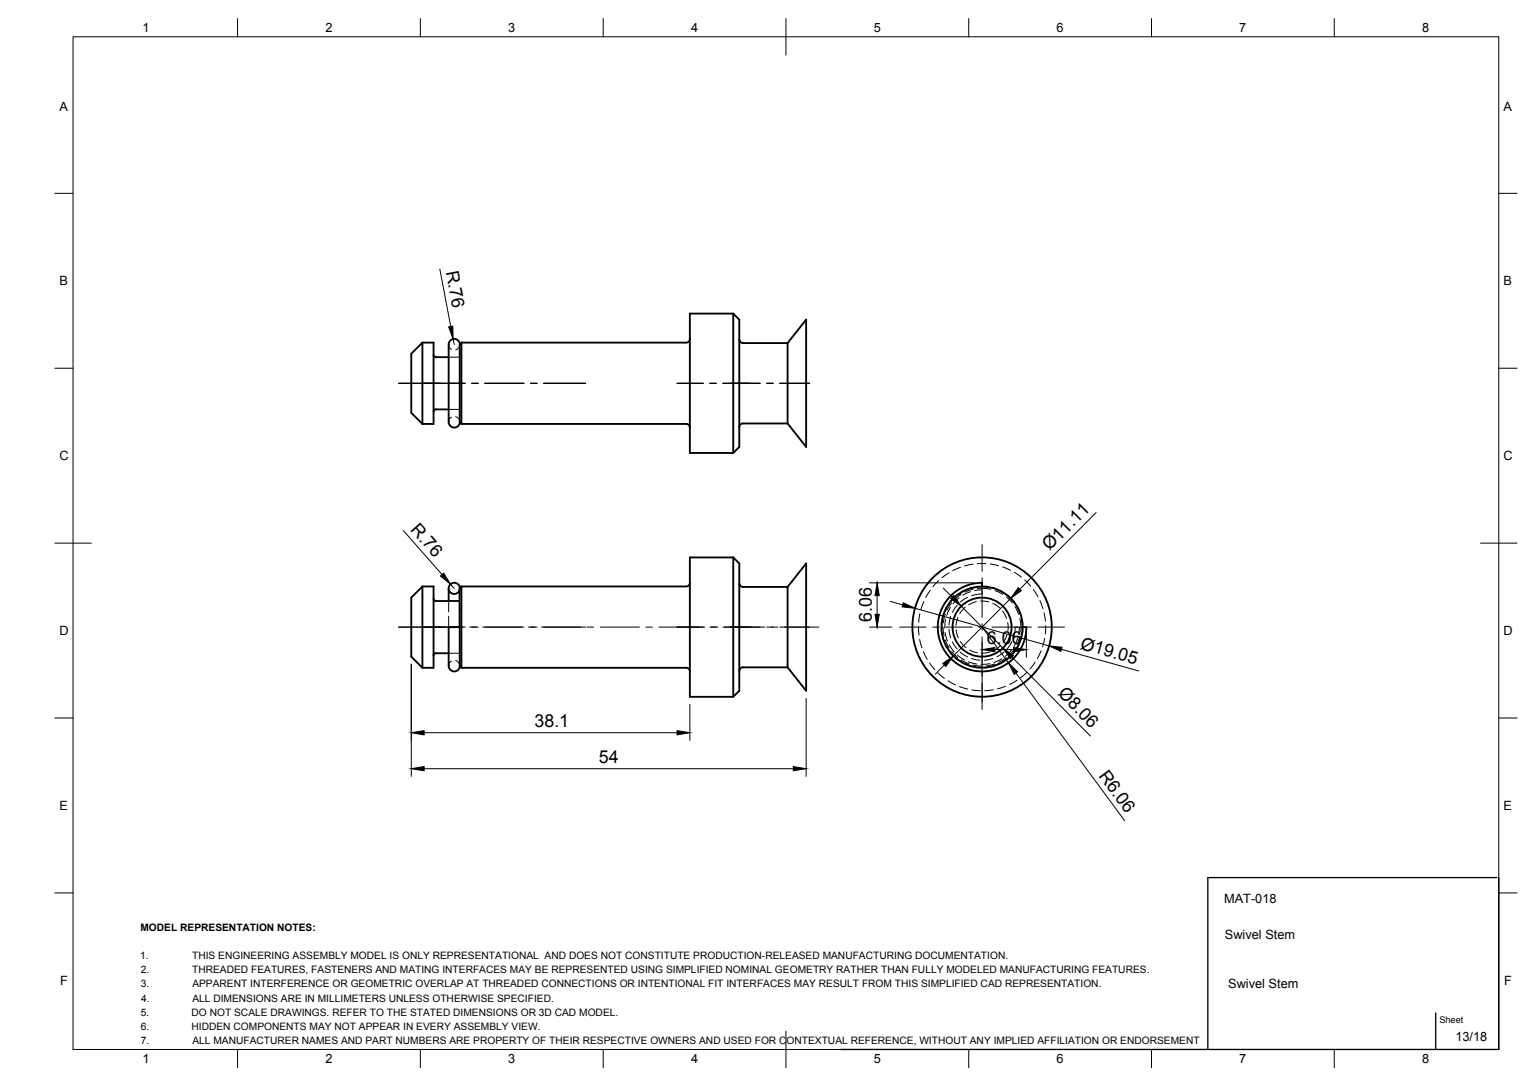
ISO-10303-21;
HEADER;
/* Generated by software containing ST-Developer
 * from STEP Tools, Inc. (www.steptools.com) 
 */

FILE_DESCRIPTION(
/* description */ ('STEP AP214'),
/* implementation_level */ '2;1');

FILE_NAME(
/* name */ 'Swivel Stem.step',
/* time_stamp */ '2026-11-14T06:16:09-08:00',
/* author */ (''),
/* organization */ (''),
/* preprocessor_version */ 'ST-DEVELOPER v20.2',
/* originating_system */ 'Autodesk Translation Framework v15.17.0.0',
/* authorisation */ '');

FILE_SCHEMA (('AUTOMOTIVE_DESIGN { 1 0 10303 214 3 1 1 }'));
ENDSEC;

DATA;
#10=MECHANICAL_DESIGN_GEOMETRIC_PRESENTATION_REPRESENTATION('',(#357),#18006);
#137=CONICAL_SURFACE('',#10642,5.30225,0.78539816339744);
#138=CONICAL_SURFACE('',#10645,4.03225,0.785398163397449);
#139=CONICAL_SURFACE('',#10665,9.525,0.785398163397447);
#140=CONICAL_SURFACE('',#10673,5.4991,0.899938860194128);
#248=TOROIDAL_SURFACE('',#10636,5.2959,0.762);
#249=TOROIDAL_SURFACE('',#10650,3.8862,0.3175);
#250=TOROIDAL_SURFACE('',#10658,6.06425,0.508);
#251=TOROIDAL_SURFACE('',#10667,6.0071,0.508);
#325=SHAPE_REPRESENTATION_RELATIONSHIP('SRR','None',#18083,#341);
#341=ADVANCED_BREP_SHAPE_REPRESENTATION('',(#373),#18000);
#357=STYLED_ITEM('',(#18170),#373);
#373=MANIFOLD_SOLID_BREP('Body1',#9566);
#478=FACE_BOUND('',#2020,.T.);
#479=FACE_BOUND('',#2022,.T.);
#480=FACE_BOUND('',#2024,.T.);
#481=FACE_BOUND('',#2027,.T.);
#805=PLANE('',#10675);
#806=PLANE('',#10676);
#807=PLANE('',#10677);
#808=PLANE('',#10678);
#809=PLANE('',#10679);
#810=PLANE('',#10680);
#811=PLANE('',#10681);
#812=PLANE('',#10682);
#1328=FACE_OUTER_BOUND('',#2003,.T.);
#1329=FACE_OUTER_BOUND('',#2004,.T.);
#1330=FACE_OUTER_BOUND('',#2005,.T.);
#1331=FACE_OUTER_BOUND('',#2006,.T.);
#1332=FACE_OUTER_BOUND('',#2007,.T.);
#1333=FACE_OUTER_BOUND('',#2008,.T.);
#1334=FACE_OUTER_BOUND('',#2009,.T.);
#1335=FACE_OUTER_BOUND('',#2010,.T.);
#1336=FACE_OUTER_BOUND('',#2011,.T.);
#1337=FACE_OUTER_BOUND('',#2012,.T.);
#1338=FACE_OUTER_BOUND('',#2013,.T.);
#1339=FACE_OUTER_BOUND('',#2014,.T.);
#1340=FACE_OUTER_BOUND('',#2015,.T.);
#1341=FACE_OUTER_BOUND('',#2016,.T.);
#1342=FACE_OUTER_BOUND('',#2017,.T.);
#1343=FACE_OUTER_BOUND('',#2018,.T.);
#1344=FACE_OUTER_BOUND('',#2019,.T.);
#1345=FACE_OUTER_BOUND('',#2021,.T.);
#1346=FACE_OUTER_BOUND('',#2023,.T.);
#1347=FACE_OUTER_BOUND('',#2025,.T.);
#1348=FACE_OUTER_BOUND('',#2026,.T.);
#2003=EDGE_LOOP('',(#8466,#8467,#8468,#8469,#8470));
#2004=EDGE_LOOP('',(#8471,#8472,#8473,#8474,#8475,#8476,#8477,#8478));
#2005=EDGE_LOOP('',(#8479,#8480,#8481,#8482));
#2006=EDGE_LOOP('',(#8483,#8484,#8485,#8486));
#2007=EDGE_LOOP('',(#8487,#8488,#8489,#8490));
#2008=EDGE_LOOP('',(#8491,#8492,#8493,#8494));
#2009=EDGE_LOOP('',(#8495,#8496,#8497,#8498));
#2010=EDGE_LOOP('',(#8499,#8500,#8501,#8502));
#2011=EDGE_LOOP('',(#8503,#8504,#8505,#8506,#8507));
#2012=EDGE_LOOP('',(#8508,#8509,#8510,#8511,#8512));
#2013=EDGE_LOOP('',(#8513,#8514,#8515,#8516));
#2014=EDGE_LOOP('',(#8517,#8518,#8519,#8520));
#2015=EDGE_LOOP('',(#8521,#8522,#8523,#8524));
#2016=EDGE_LOOP('',(#8525,#8526,#8527));
#2017=EDGE_LOOP('',(#8528,#8529,#8530));
#2018=EDGE_LOOP('',(#8531));
#2019=EDGE_LOOP('',(#8532));
#2020=EDGE_LOOP('',(#8533));
#2021=EDGE_LOOP('',(#8534));
#2022=EDGE_LOOP('',(#8535));
#2023=EDGE_LOOP('',(#8536));
#2024=EDGE_LOOP('',(#8537));
#2025=EDGE_LOOP('',(#8538));
#2026=EDGE_LOOP('',(#8539,#8540,#8541,#8542));
#2027=EDGE_LOOP('',(#8543));
#2779=LINE('',#17587,#3503);
#2780=LINE('',#17589,#3504);
#2781=LINE('',#17592,#3505);
#2782=LINE('',#17597,#3506);
#2783=LINE('',#17602,#3507);
#2784=LINE('',#17612,#3508);
#2785=LINE('',#17616,#3509);
#2786=LINE('',#17627,#3510);
#2787=LINE('',#17631,#3511);
#2788=LINE('',#17642,#3512);
#2789=LINE('',#17646,#3513);
#2790=LINE('',#17648,#3514);
#2791=LINE('',#17650,#3515);
#3503=VECTOR('',#13314,5.30225);
#3504=VECTOR('',#13315,1000.);
#3505=VECTOR('',#13318,1000.);
#3506=VECTOR('',#13323,4.03225);
#3507=VECTOR('',#13330,5.55625);
#3508=VECTOR('',#13343,3.5687);
#3509=VECTOR('',#13348,5.55625);
#3510=VECTOR('',#13361,9.525);
#3511=VECTOR('',#13366,9.525);
#3512=VECTOR('',#13381,5.4991);
#3513=VECTOR('',#13386,5.4991);
#3514=VECTOR('',#13389,1000.);
#3515=VECTOR('',#13392,1000.);
#3903=CIRCLE('',#10637,0.762);
#3904=CIRCLE('',#10638,5.32701449118557);
#3905=CIRCLE('',#10639,5.32701449118557);
#3906=CIRCLE('',#10640,0.762);
#3907=CIRCLE('',#10641,5.10079889800413);
#3908=CIRCLE('',#10643,5.55625);
#3909=CIRCLE('',#10644,5.30225);
#3910=CIRCLE('',#10646,5.55625);
#3911=CIRCLE('',#10647,4.03225);
#3912=CIRCLE('',#10649,5.55625);
#3913=CIRCLE('',#10651,3.5687);
#3914=CIRCLE('',#10652,0.3175);
#3915=CIRCLE('',#10653,3.8862);
#3916=CIRCLE('',#10655,3.5687);
#3917=CIRCLE('',#10657,5.55625);
#3918=CIRCLE('',#10659,6.06425);
#3919=CIRCLE('',#10660,0.508);
#3920=CIRCLE('',#10662,9.525);
#3921=CIRCLE('',#10663,9.525);
#3922=CIRCLE('',#10664,9.525);
#3923=CIRCLE('',#10666,8.6995);
#3924=CIRCLE('',#10668,5.4991);
#3925=CIRCLE('',#10669,0.508);
#3926=CIRCLE('',#10670,6.0071);
#3927=CIRCLE('',#10672,5.4991);
#3928=CIRCLE('',#10674,8.6995);
#4716=VERTEX_POINT('',#17574);
#4717=VERTEX_POINT('',#17575);
#4718=VERTEX_POINT('',#17577);
#4719=VERTEX_POINT('',#17579);
#4720=VERTEX_POINT('',#17581);
#4721=VERTEX_POINT('',#17585);
#4722=VERTEX_POINT('',#17588);
#4723=VERTEX_POINT('',#17590);
#4724=VERTEX_POINT('',#17594);
#4725=VERTEX_POINT('',#17596);
#4726=VERTEX_POINT('',#17600);
#4727=VERTEX_POINT('',#17604);
#4728=VERTEX_POINT('',#17606);
#4729=VERTEX_POINT('',#17610);
#4730=VERTEX_POINT('',#17614);
#4731=VERTEX_POINT('',#17618);
#4732=VERTEX_POINT('',#17622);
#4733=VERTEX_POINT('',#17623);
#4734=VERTEX_POINT('',#17626);
#4735=VERTEX_POINT('',#17630);
#4736=VERTEX_POINT('',#17634);
#4737=VERTEX_POINT('',#17636);
#4738=VERTEX_POINT('',#17640);
#4739=VERTEX_POINT('',#17644);
#5981=EDGE_CURVE('',#4716,#4717,#3903,.T.);
#5982=EDGE_CURVE('',#4718,#4716,#3904,.T.);
#5983=EDGE_CURVE('',#4719,#4718,#3905,.T.);
#5984=EDGE_CURVE('',#4719,#4720,#3906,.T.);
#5985=EDGE_CURVE('',#4717,#4720,#3907,.T.);
#5986=EDGE_CURVE('',#4721,#4721,#3908,.T.);
#5987=EDGE_CURVE('',#4721,#4718,#2779,.T.);
#5988=EDGE_CURVE('',#4716,#4722,#2780,.T.);
#5989=EDGE_CURVE('',#4722,#4723,#3909,.T.);
#5990=EDGE_CURVE('',#4719,#4723,#2781,.T.);
#5991=EDGE_CURVE('',#4724,#4724,#3910,.T.);
#5992=EDGE_CURVE('',#4724,#4725,#2782,.T.);
#5993=EDGE_CURVE('',#4725,#4725,#3911,.T.);
#5994=EDGE_CURVE('',#4726,#4726,#3912,.T.);
#5995=EDGE_CURVE('',#4726,#4724,#2783,.T.);
#5996=EDGE_CURVE('',#4727,#4727,#3913,.T.);
#5997=EDGE_CURVE('',#4727,#4728,#3914,.T.);
#5998=EDGE_CURVE('',#4728,#4728,#3915,.T.);
#5999=EDGE_CURVE('',#4729,#4729,#3916,.T.);
#6000=EDGE_CURVE('',#4729,#4727,#2784,.T.);
#6001=EDGE_CURVE('',#4730,#4730,#3917,.T.);
#6002=EDGE_CURVE('',#4730,#4721,#2785,.T.);
#6003=EDGE_CURVE('',#4731,#4731,#3918,.T.);
#6004=EDGE_CURVE('',#4731,#4730,#3919,.T.);
#6005=EDGE_CURVE('',#4732,#4733,#3920,.T.);
#6006=EDGE_CURVE('',#4733,#4732,#3921,.T.);
#6007=EDGE_CURVE('',#4733,#4734,#2786,.T.);
#6008=EDGE_CURVE('',#4734,#4734,#3922,.T.);
#6009=EDGE_CURVE('',#4732,#4735,#2787,.T.);
#6010=EDGE_CURVE('',#4735,#4735,#3923,.T.);
#6011=EDGE_CURVE('',#4736,#4736,#3924,.T.);
#6012=EDGE_CURVE('',#4736,#4737,#3925,.T.);
#6013=EDGE_CURVE('',#4737,#4737,#3926,.T.);
#6014=EDGE_CURVE('',#4738,#4738,#3927,.T.);
#6015=EDGE_CURVE('',#4738,#4736,#2788,.T.);
#6016=EDGE_CURVE('',#4739,#4739,#3928,.T.);
#6017=EDGE_CURVE('',#4739,#4738,#2789,.T.);
#6018=EDGE_CURVE('',#4722,#4717,#2790,.T.);
#6019=EDGE_CURVE('',#4723,#4720,#2791,.T.);
#8466=ORIENTED_EDGE('',*,*,#5981,.F.);
#8467=ORIENTED_EDGE('',*,*,#5982,.F.);
#8468=ORIENTED_EDGE('',*,*,#5983,.F.);
#8469=ORIENTED_EDGE('',*,*,#5984,.T.);
#8470=ORIENTED_EDGE('',*,*,#5985,.F.);
#8471=ORIENTED_EDGE('',*,*,#5986,.F.);
#8472=ORIENTED_EDGE('',*,*,#5987,.T.);
#8473=ORIENTED_EDGE('',*,*,#5982,.T.);
#8474=ORIENTED_EDGE('',*,*,#5988,.T.);
#8475=ORIENTED_EDGE('',*,*,#5989,.T.);
#8476=ORIENTED_EDGE('',*,*,#5990,.F.);
#8477=ORIENTED_EDGE('',*,*,#5983,.T.);
#8478=ORIENTED_EDGE('',*,*,#5987,.F.);
#8479=ORIENTED_EDGE('',*,*,#5991,.F.);
#8480=ORIENTED_EDGE('',*,*,#5992,.T.);
#8481=ORIENTED_EDGE('',*,*,#5993,.T.);
#8482=ORIENTED_EDGE('',*,*,#5992,.F.);
#8483=ORIENTED_EDGE('',*,*,#5994,.F.);
#8484=ORIENTED_EDGE('',*,*,#5995,.T.);
#8485=ORIENTED_EDGE('',*,*,#5991,.T.);
#8486=ORIENTED_EDGE('',*,*,#5995,.F.);
#8487=ORIENTED_EDGE('',*,*,#5996,.F.);
#8488=ORIENTED_EDGE('',*,*,#5997,.T.);
#8489=ORIENTED_EDGE('',*,*,#5998,.T.);
#8490=ORIENTED_EDGE('',*,*,#5997,.F.);
#8491=ORIENTED_EDGE('',*,*,#5999,.F.);
#8492=ORIENTED_EDGE('',*,*,#6000,.T.);
#8493=ORIENTED_EDGE('',*,*,#5996,.T.);
#8494=ORIENTED_EDGE('',*,*,#6000,.F.);
#8495=ORIENTED_EDGE('',*,*,#6001,.F.);
#8496=ORIENTED_EDGE('',*,*,#6002,.T.);
#8497=ORIENTED_EDGE('',*,*,#5986,.T.);
#8498=ORIENTED_EDGE('',*,*,#6002,.F.);
#8499=ORIENTED_EDGE('',*,*,#6003,.F.);
#8500=ORIENTED_EDGE('',*,*,#6004,.T.);
#8501=ORIENTED_EDGE('',*,*,#6001,.T.);
#8502=ORIENTED_EDGE('',*,*,#6004,.F.);
#8503=ORIENTED_EDGE('',*,*,#6005,.F.);
#8504=ORIENTED_EDGE('',*,*,#6006,.F.);
#8505=ORIENTED_EDGE('',*,*,#6007,.T.);
#8506=ORIENTED_EDGE('',*,*,#6008,.T.);
#8507=ORIENTED_EDGE('',*,*,#6007,.F.);
#8508=ORIENTED_EDGE('',*,*,#6005,.T.);
#8509=ORIENTED_EDGE('',*,*,#6006,.T.);
#8510=ORIENTED_EDGE('',*,*,#6009,.T.);
#8511=ORIENTED_EDGE('',*,*,#6010,.F.);
#8512=ORIENTED_EDGE('',*,*,#6009,.F.);
#8513=ORIENTED_EDGE('',*,*,#6011,.F.);
#8514=ORIENTED_EDGE('',*,*,#6012,.T.);
#8515=ORIENTED_EDGE('',*,*,#6013,.T.);
#8516=ORIENTED_EDGE('',*,*,#6012,.F.);
#8517=ORIENTED_EDGE('',*,*,#6014,.F.);
#8518=ORIENTED_EDGE('',*,*,#6015,.T.);
#8519=ORIENTED_EDGE('',*,*,#6011,.T.);
#8520=ORIENTED_EDGE('',*,*,#6015,.F.);
#8521=ORIENTED_EDGE('',*,*,#6016,.F.);
#8522=ORIENTED_EDGE('',*,*,#6017,.T.);
#8523=ORIENTED_EDGE('',*,*,#6014,.T.);
#8524=ORIENTED_EDGE('',*,*,#6017,.F.);
#8525=ORIENTED_EDGE('',*,*,#6018,.F.);
#8526=ORIENTED_EDGE('',*,*,#5988,.F.);
#8527=ORIENTED_EDGE('',*,*,#5981,.T.);
#8528=ORIENTED_EDGE('',*,*,#5990,.T.);
#8529=ORIENTED_EDGE('',*,*,#6019,.T.);
#8530=ORIENTED_EDGE('',*,*,#5984,.F.);
#8531=ORIENTED_EDGE('',*,*,#6016,.T.);
#8532=ORIENTED_EDGE('',*,*,#6010,.T.);
#8533=ORIENTED_EDGE('',*,*,#6013,.F.);
#8534=ORIENTED_EDGE('',*,*,#6008,.F.);
#8535=ORIENTED_EDGE('',*,*,#6003,.T.);
#8536=ORIENTED_EDGE('',*,*,#5994,.T.);
#8537=ORIENTED_EDGE('',*,*,#5998,.F.);
#8538=ORIENTED_EDGE('',*,*,#5993,.F.);
#8539=ORIENTED_EDGE('',*,*,#6019,.F.);
#8540=ORIENTED_EDGE('',*,*,#5989,.F.);
#8541=ORIENTED_EDGE('',*,*,#6018,.T.);
#8542=ORIENTED_EDGE('',*,*,#5985,.T.);
#8543=ORIENTED_EDGE('',*,*,#5999,.T.);
#8963=CYLINDRICAL_SURFACE('',#10648,5.55625);
#8964=CYLINDRICAL_SURFACE('',#10654,3.5687);
#8965=CYLINDRICAL_SURFACE('',#10656,5.55625);
#8966=CYLINDRICAL_SURFACE('',#10661,9.525);
#8967=CYLINDRICAL_SURFACE('',#10671,5.4991);
#9467=ADVANCED_FACE('',(#1328),#248,.T.);
#9468=ADVANCED_FACE('',(#1329),#137,.T.);
#9469=ADVANCED_FACE('',(#1330),#138,.T.);
#9470=ADVANCED_FACE('',(#1331),#8963,.T.);
#9471=ADVANCED_FACE('',(#1332),#249,.F.);
#9472=ADVANCED_FACE('',(#1333),#8964,.T.);
#9473=ADVANCED_FACE('',(#1334),#8965,.T.);
#9474=ADVANCED_FACE('',(#1335),#250,.F.);
#9475=ADVANCED_FACE('',(#1336),#8966,.T.);
#9476=ADVANCED_FACE('',(#1337),#139,.T.);
#9477=ADVANCED_FACE('',(#1338),#251,.F.);
#9478=ADVANCED_FACE('',(#1339),#8967,.T.);
#9479=ADVANCED_FACE('',(#1340),#140,.T.);
#9480=ADVANCED_FACE('',(#1341),#805,.T.);
#9481=ADVANCED_FACE('',(#1342),#806,.F.);
#9482=ADVANCED_FACE('',(#1343),#807,.F.);
#9483=ADVANCED_FACE('',(#1344,#478),#808,.F.);
#9484=ADVANCED_FACE('',(#1345,#479),#809,.F.);
#9485=ADVANCED_FACE('',(#1346,#480),#810,.F.);
#9486=ADVANCED_FACE('',(#1347),#811,.F.);
#9487=ADVANCED_FACE('',(#1348,#481),#812,.F.);
#9566=CLOSED_SHELL('',(#9467,#9468,#9469,#9470,#9471,#9472,#9473,#9474,
#9475,#9476,#9477,#9478,#9479,#9480,#9481,#9482,#9483,#9484,#9485,#9486,
#9487));
#10635=AXIS2_PLACEMENT_3D('',#17572,#13296,#13297);
#10636=AXIS2_PLACEMENT_3D('',#17573,#13298,#13299);
#10637=AXIS2_PLACEMENT_3D('',#17576,#13300,#13301);
#10638=AXIS2_PLACEMENT_3D('',#17578,#13302,#13303);
#10639=AXIS2_PLACEMENT_3D('',#17580,#13304,#13305);
#10640=AXIS2_PLACEMENT_3D('',#17582,#13306,#13307);
#10641=AXIS2_PLACEMENT_3D('',#17583,#13308,#13309);
#10642=AXIS2_PLACEMENT_3D('',#17584,#13310,#13311);
#10643=AXIS2_PLACEMENT_3D('',#17586,#13312,#13313);
#10644=AXIS2_PLACEMENT_3D('',#17591,#13316,#13317);
#10645=AXIS2_PLACEMENT_3D('',#17593,#13319,#13320);
#10646=AXIS2_PLACEMENT_3D('',#17595,#13321,#13322);
#10647=AXIS2_PLACEMENT_3D('',#17598,#13324,#13325);
#10648=AXIS2_PLACEMENT_3D('',#17599,#13326,#13327);
#10649=AXIS2_PLACEMENT_3D('',#17601,#13328,#13329);
#10650=AXIS2_PLACEMENT_3D('',#17603,#13331,#13332);
#10651=AXIS2_PLACEMENT_3D('',#17605,#13333,#13334);
#10652=AXIS2_PLACEMENT_3D('',#17607,#13335,#13336);
#10653=AXIS2_PLACEMENT_3D('',#17608,#13337,#13338);
#10654=AXIS2_PLACEMENT_3D('',#17609,#13339,#13340);
#10655=AXIS2_PLACEMENT_3D('',#17611,#13341,#13342);
#10656=AXIS2_PLACEMENT_3D('',#17613,#13344,#13345);
#10657=AXIS2_PLACEMENT_3D('',#17615,#13346,#13347);
#10658=AXIS2_PLACEMENT_3D('',#17617,#13349,#13350);
#10659=AXIS2_PLACEMENT_3D('',#17619,#13351,#13352);
#10660=AXIS2_PLACEMENT_3D('',#17620,#13353,#13354);
#10661=AXIS2_PLACEMENT_3D('',#17621,#13355,#13356);
#10662=AXIS2_PLACEMENT_3D('',#17624,#13357,#13358);
#10663=AXIS2_PLACEMENT_3D('',#17625,#13359,#13360);
#10664=AXIS2_PLACEMENT_3D('',#17628,#13362,#13363);
#10665=AXIS2_PLACEMENT_3D('',#17629,#13364,#13365);
#10666=AXIS2_PLACEMENT_3D('',#17632,#13367,#13368);
#10667=AXIS2_PLACEMENT_3D('',#17633,#13369,#13370);
#10668=AXIS2_PLACEMENT_3D('',#17635,#13371,#13372);
#10669=AXIS2_PLACEMENT_3D('',#17637,#13373,#13374);
#10670=AXIS2_PLACEMENT_3D('',#17638,#13375,#13376);
#10671=AXIS2_PLACEMENT_3D('',#17639,#13377,#13378);
#10672=AXIS2_PLACEMENT_3D('',#17641,#13379,#13380);
#10673=AXIS2_PLACEMENT_3D('',#17643,#13382,#13383);
#10674=AXIS2_PLACEMENT_3D('',#17645,#13384,#13385);
#10675=AXIS2_PLACEMENT_3D('',#17647,#13387,#13388);
#10676=AXIS2_PLACEMENT_3D('',#17649,#13390,#13391);
#10677=AXIS2_PLACEMENT_3D('',#17651,#13393,#13394);
#10678=AXIS2_PLACEMENT_3D('',#17652,#13395,#13396);
#10679=AXIS2_PLACEMENT_3D('',#17653,#13397,#13398);
#10680=AXIS2_PLACEMENT_3D('',#17654,#13399,#13400);
#10681=AXIS2_PLACEMENT_3D('',#17655,#13401,#13402);
#10682=AXIS2_PLACEMENT_3D('',#17656,#13403,#13404);
#13296=DIRECTION('axis',(0.,0.,1.));
#13297=DIRECTION('refdir',(1.,0.,0.));
#13298=DIRECTION('center_axis',(1.,0.,0.));
#13299=DIRECTION('ref_axis',(0.,0.,-1.));
#13300=DIRECTION('center_axis',(0.,-0.707106781186547,0.707106781186548));
#13301=DIRECTION('ref_axis',(1.,0.,0.));
#13302=DIRECTION('center_axis',(1.,1.3055303676213E-17,0.));
#13303=DIRECTION('ref_axis',(1.3055303676213E-17,-1.,0.));
#13304=DIRECTION('center_axis',(1.,1.3055303676213E-17,0.));
#13305=DIRECTION('ref_axis',(1.3055303676213E-17,-1.,0.));
#13306=DIRECTION('center_axis',(0.,-0.707106781186547,-0.707106781186548));
#13307=DIRECTION('ref_axis',(1.,0.,0.));
#13308=DIRECTION('center_axis',(-1.,-1.3055303676213E-17,0.));
#13309=DIRECTION('ref_axis',(1.3055303676213E-17,-1.,0.));
#13310=DIRECTION('center_axis',(1.,1.3055303676213E-17,0.));
#13311=DIRECTION('ref_axis',(-1.3055303676213E-17,1.,0.));
#13312=DIRECTION('center_axis',(1.,1.3055303676213E-17,0.));
#13313=DIRECTION('ref_axis',(-1.3055303676213E-17,1.,0.));
#13314=DIRECTION('',(-0.707106781186553,0.707106781186542,8.65956056235486E-17));
#13315=DIRECTION('',(-0.707106781186551,-0.499999999999998,-0.499999999999998));
#13316=DIRECTION('center_axis',(1.,1.3055303676213E-17,0.));
#13317=DIRECTION('ref_axis',(-1.3055303676213E-17,1.,0.));
#13318=DIRECTION('',(-0.707106781186551,0.499999999999998,-0.499999999999998));
#13319=DIRECTION('center_axis',(1.,1.3055303676213E-17,0.));
#13320=DIRECTION('ref_axis',(-1.3055303676213E-17,1.,0.));
#13321=DIRECTION('center_axis',(1.,1.3055303676213E-17,0.));
#13322=DIRECTION('ref_axis',(-1.3055303676213E-17,1.,0.));
#13323=DIRECTION('',(-0.707106781186547,0.707106781186548,8.65956056235494E-17));
#13324=DIRECTION('center_axis',(1.,1.3055303676213E-17,0.));
#13325=DIRECTION('ref_axis',(-1.3055303676213E-17,1.,0.));
#13326=DIRECTION('center_axis',(1.,1.3055303676213E-17,0.));
#13327=DIRECTION('ref_axis',(-1.3055303676213E-17,1.,0.));
#13328=DIRECTION('center_axis',(1.,1.3055303676213E-17,0.));
#13329=DIRECTION('ref_axis',(-1.3055303676213E-17,1.,0.));
#13330=DIRECTION('',(-1.,-1.3055303676213E-17,0.));
#13331=DIRECTION('center_axis',(1.,1.3055303676213E-17,0.));
#13332=DIRECTION('ref_axis',(0.,1.,0.));
#13333=DIRECTION('center_axis',(1.,1.3055303676213E-17,0.));
#13334=DIRECTION('ref_axis',(-1.3055303676213E-17,1.,0.));
#13335=DIRECTION('center_axis',(1.59881358589709E-33,-1.22464679914735E-16,
1.));
#13336=DIRECTION('ref_axis',(0.,-1.,-1.22464679914735E-16));
#13337=DIRECTION('center_axis',(1.,1.3055303676213E-17,0.));
#13338=DIRECTION('ref_axis',(-1.3055303676213E-17,1.,0.));
#13339=DIRECTION('center_axis',(1.,1.3055303676213E-17,0.));
#13340=DIRECTION('ref_axis',(-1.3055303676213E-17,1.,0.));
#13341=DIRECTION('center_axis',(1.,1.3055303676213E-17,0.));
#13342=DIRECTION('ref_axis',(-1.3055303676213E-17,1.,0.));
#13343=DIRECTION('',(-1.,-1.3055303676213E-17,0.));
#13344=DIRECTION('center_axis',(1.,1.3055303676213E-17,0.));
#13345=DIRECTION('ref_axis',(-1.3055303676213E-17,1.,0.));
#13346=DIRECTION('center_axis',(1.,1.3055303676213E-17,0.));
#13347=DIRECTION('ref_axis',(-1.3055303676213E-17,1.,0.));
#13348=DIRECTION('',(-1.,-1.3055303676213E-17,0.));
#13349=DIRECTION('center_axis',(1.,1.3055303676213E-17,0.));
#13350=DIRECTION('ref_axis',(0.,1.,0.));
#13351=DIRECTION('center_axis',(1.,1.3055303676213E-17,0.));
#13352=DIRECTION('ref_axis',(-1.3055303676213E-17,1.,0.));
#13353=DIRECTION('center_axis',(1.59881358589709E-33,-1.22464679914735E-16,
1.));
#13354=DIRECTION('ref_axis',(0.,-1.,-1.22464679914735E-16));
#13355=DIRECTION('center_axis',(1.,1.3055303676213E-17,0.));
#13356=DIRECTION('ref_axis',(-1.3055303676213E-17,1.,0.));
#13357=DIRECTION('center_axis',(1.,1.3055303676213E-17,0.));
#13358=DIRECTION('ref_axis',(-1.3055303676213E-17,1.,0.));
#13359=DIRECTION('center_axis',(1.,1.3055303676213E-17,0.));
#13360=DIRECTION('ref_axis',(-1.3055303676213E-17,1.,0.));
#13361=DIRECTION('',(-1.,-1.3055303676213E-17,0.));
#13362=DIRECTION('center_axis',(1.,1.3055303676213E-17,0.));
#13363=DIRECTION('ref_axis',(-1.3055303676213E-17,1.,0.));
#13364=DIRECTION('center_axis',(-1.,-1.3055303676213E-17,0.));
#13365=DIRECTION('ref_axis',(1.3055303676213E-17,-1.,0.));
#13366=DIRECTION('',(0.707106781186549,-0.707106781186547,8.65956056235492E-17));
#13367=DIRECTION('center_axis',(1.,1.3055303676213E-17,0.));
#13368=DIRECTION('ref_axis',(-1.3055303676213E-17,1.,0.));
#13369=DIRECTION('center_axis',(1.,1.3055303676213E-17,0.));
#13370=DIRECTION('ref_axis',(0.,1.,0.));
#13371=DIRECTION('center_axis',(1.,1.3055303676213E-17,0.));
#13372=DIRECTION('ref_axis',(-1.3055303676213E-17,1.,0.));
#13373=DIRECTION('center_axis',(1.59881358589709E-33,-1.22464679914735E-16,
1.));
#13374=DIRECTION('ref_axis',(0.,-1.,-1.22464679914735E-16));
#13375=DIRECTION('center_axis',(1.,1.3055303676213E-17,0.));
#13376=DIRECTION('ref_axis',(-1.3055303676213E-17,1.,0.));
#13377=DIRECTION('center_axis',(1.,1.3055303676213E-17,0.));
#13378=DIRECTION('ref_axis',(-1.3055303676213E-17,1.,0.));
#13379=DIRECTION('center_axis',(1.,1.3055303676213E-17,0.));
#13380=DIRECTION('ref_axis',(-1.3055303676213E-17,1.,0.));
#13381=DIRECTION('',(-1.,-1.3055303676213E-17,0.));
#13382=DIRECTION('center_axis',(1.,1.3055303676213E-17,0.));
#13383=DIRECTION('ref_axis',(-1.3055303676213E-17,1.,0.));
#13384=DIRECTION('center_axis',(1.,1.3055303676213E-17,0.));
#13385=DIRECTION('ref_axis',(-1.3055303676213E-17,1.,0.));
#13386=DIRECTION('',(-0.621657859564011,0.783288903050651,9.59252247928621E-17));
#13387=DIRECTION('center_axis',(0.,-0.707106781186547,0.707106781186548));
#13388=DIRECTION('ref_axis',(-1.,0.,0.));
#13389=DIRECTION('',(9.2314937598999E-18,-0.707106781186548,-0.707106781186547));
#13390=DIRECTION('center_axis',(0.,-0.707106781186547,-0.707106781186548));
#13391=DIRECTION('ref_axis',(0.,-0.707106781186548,0.707106781186547));
#13392=DIRECTION('',(-9.2314937598999E-18,0.707106781186548,-0.707106781186547));
#13393=DIRECTION('center_axis',(-1.,-1.3055303676213E-17,0.));
#13394=DIRECTION('ref_axis',(-1.3055303676213E-17,1.,0.));
#13395=DIRECTION('center_axis',(-1.,-1.3055303676213E-17,0.));
#13396=DIRECTION('ref_axis',(-1.3055303676213E-17,1.,0.));
#13397=DIRECTION('center_axis',(1.,1.3055303676213E-17,0.));
#13398=DIRECTION('ref_axis',(-1.3055303676213E-17,1.,0.));
#13399=DIRECTION('center_axis',(-1.,-1.3055303676213E-17,0.));
#13400=DIRECTION('ref_axis',(-1.3055303676213E-17,1.,0.));
#13401=DIRECTION('center_axis',(1.,1.3055303676213E-17,0.));
#13402=DIRECTION('ref_axis',(-1.3055303676213E-17,1.,0.));
#13403=DIRECTION('center_axis',(1.,1.3055303676213E-17,0.));
#13404=DIRECTION('ref_axis',(-1.3055303676213E-17,1.,0.));
#17572=CARTESIAN_POINT('',(0.,0.,0.));
#17573=CARTESIAN_POINT('Origin',(5.8674,0.,0.));
#17574=CARTESIAN_POINT('',(6.62876449118558,3.76676807019632,3.76676807019632));
#17575=CARTESIAN_POINT('',(6.604,3.6068094902476,3.6068094902476));
#17576=CARTESIAN_POINT('Origin',(5.8674,3.74476680248583,3.74476680248583));
#17577=CARTESIAN_POINT('',(6.62876449118558,-5.32701449118557,-6.52371124564198E-16));
#17578=CARTESIAN_POINT('Origin',(6.62876449118558,9.93984464071305E-18,
0.));
#17579=CARTESIAN_POINT('',(6.62876449118558,-3.76676807019632,3.76676807019632));
#17580=CARTESIAN_POINT('Origin',(6.62876449118558,9.93984464071305E-18,
0.));
#17581=CARTESIAN_POINT('',(6.604,-3.6068094902476,3.6068094902476));
#17582=CARTESIAN_POINT('Origin',(5.8674,-3.74476680248583,3.74476680248583));
#17583=CARTESIAN_POINT('Origin',(6.604,9.61653668789852E-18,0.));
#17584=CARTESIAN_POINT('Origin',(6.604,8.62172254777109E-17,0.));
#17585=CARTESIAN_POINT('',(6.858,-5.55625,-6.80444377776248E-16));
#17586=CARTESIAN_POINT('Origin',(6.858,8.9533272611469E-17,0.));
#17587=CARTESIAN_POINT('',(6.604,-5.30225,-6.49338349077905E-16));
#17588=CARTESIAN_POINT('',(6.604,3.74925693054637,3.74925693054637));
#17589=CARTESIAN_POINT('',(1.30174999999991,3.23653424897184E-16,-3.06658683336675E-16));
#17590=CARTESIAN_POINT('',(6.604,-3.74925693054637,3.74925693054637));
#17591=CARTESIAN_POINT('Origin',(6.604,8.62172254777109E-17,0.));
#17592=CARTESIAN_POINT('',(1.30174999999991,1.69947415605091E-17,0.));
#17593=CARTESIAN_POINT('Origin',(0.,0.,0.));
#17594=CARTESIAN_POINT('',(1.524,-5.55625,-6.80444377776248E-16));
#17595=CARTESIAN_POINT('Origin',(1.524,1.98962828025486E-17,0.));
#17596=CARTESIAN_POINT('',(-1.58418895642851E-17,-4.03225,-4.93808205586192E-16));
#17597=CARTESIAN_POINT('',(5.26422482484099E-17,-4.03225,-4.93808205586192E-16));
#17598=CARTESIAN_POINT('Origin',(0.,0.,0.));
#17599=CARTESIAN_POINT('Origin',(54.0004,7.04991620636974E-16,0.));
#17600=CARTESIAN_POINT('',(3.048,-5.55625,-6.80444377776248E-16));
#17601=CARTESIAN_POINT('Origin',(3.048,3.97925656050972E-17,0.));
#17602=CARTESIAN_POINT('',(54.0004,-5.55625,-6.80444377776248E-16));
#17603=CARTESIAN_POINT('Origin',(3.3655,0.,0.));
#17604=CARTESIAN_POINT('',(3.3655,-3.5687,-4.37039703211716E-16));
#17605=CARTESIAN_POINT('Origin',(3.3655,4.3937624522295E-17,0.));
#17606=CARTESIAN_POINT('',(3.048,-3.8862,-4.75922239084644E-16));
#17607=CARTESIAN_POINT('Origin',(3.3655,-3.8862,-4.75922239084644E-16));
#17608=CARTESIAN_POINT('Origin',(3.048,3.97925656050972E-17,0.));
#17609=CARTESIAN_POINT('Origin',(54.0004,7.04991620636974E-16,0.));
#17610=CARTESIAN_POINT('',(6.604,-3.5687,-4.37039703211716E-16));
#17611=CARTESIAN_POINT('Origin',(6.604,8.62172254777109E-17,0.));
#17612=CARTESIAN_POINT('',(54.0004,-3.5687,-4.37039703211716E-16));
#17613=CARTESIAN_POINT('Origin',(54.0004,7.04991620636974E-16,0.));
#17614=CARTESIAN_POINT('',(37.592,-5.55625,-6.80444377776248E-16));
#17615=CARTESIAN_POINT('Origin',(37.592,4.90774975796201E-16,0.));
#17616=CARTESIAN_POINT('',(54.0004,-5.55625,-6.80444377776248E-16));
#17617=CARTESIAN_POINT('Origin',(37.592,8.67361737988404E-16,0.));
#17618=CARTESIAN_POINT('',(38.1,-6.06425,-7.42656435172934E-16));
#17619=CARTESIAN_POINT('Origin',(38.1,4.97407070063718E-16,0.));
#17620=CARTESIAN_POINT('Origin',(37.592,-6.06425,-7.42656435172934E-16));
#17621=CARTESIAN_POINT('Origin',(54.0004,7.04991620636974E-16,0.));
#17622=CARTESIAN_POINT('',(44.0309,9.525,1.16647607618785E-15));
#17623=CARTESIAN_POINT('',(44.0309,-9.525,-1.16647607618785E-15));
#17624=CARTESIAN_POINT('Origin',(44.0309,5.74836770636969E-16,0.));
#17625=CARTESIAN_POINT('Origin',(44.0309,5.74836770636969E-16,0.));
#17626=CARTESIAN_POINT('',(38.1,-9.525,-1.16647607618785E-15));
#17627=CARTESIAN_POINT('',(54.0004,-9.525,-1.16647607618785E-15));
#17628=CARTESIAN_POINT('Origin',(38.1,4.97407070063718E-16,0.));
#17629=CARTESIAN_POINT('Origin',(44.0309,5.74836770636969E-16,0.));
#17630=CARTESIAN_POINT('',(44.8564,8.6995,-1.06538148291824E-15));
#17631=CARTESIAN_POINT('',(44.0309,9.525,-1.16647607618785E-15));
#17632=CARTESIAN_POINT('Origin',(44.8564,5.85613923821682E-16,0.));
#17633=CARTESIAN_POINT('Origin',(45.3644,8.67361737988404E-16,0.));
#17634=CARTESIAN_POINT('',(45.3644,-5.4991,-6.73445521319121E-16));
#17635=CARTESIAN_POINT('Origin',(45.3644,5.92246018089199E-16,0.));
#17636=CARTESIAN_POINT('',(44.8564,-6.0071,-7.35657578715807E-16));
#17637=CARTESIAN_POINT('Origin',(45.3644,-6.0071,-7.35657578715806E-16));
#17638=CARTESIAN_POINT('Origin',(44.8564,5.85613923821682E-16,0.));
#17639=CARTESIAN_POINT('Origin',(54.0004,7.04991620636974E-16,0.));
#17640=CARTESIAN_POINT('',(51.4604,-5.4991,-6.73445521319121E-16));
#17641=CARTESIAN_POINT('Origin',(51.4604,6.71831149299393E-16,0.));
#17642=CARTESIAN_POINT('',(54.0004,-5.4991,-6.73445521319121E-16));
#17643=CARTESIAN_POINT('Origin',(51.4604,6.71831149299393E-16,0.));
#17644=CARTESIAN_POINT('',(54.0004,-8.6995,-1.06538148291824E-15));
#17645=CARTESIAN_POINT('Origin',(54.0004,7.04991620636974E-16,0.));
#17646=CARTESIAN_POINT('',(51.4604,-5.4991,-6.73445521319121E-16));
#17647=CARTESIAN_POINT('Origin',(5.8674,3.74476680248583,3.74476680248583));
#17648=CARTESIAN_POINT('',(6.604,1.78435,1.78435));
#17649=CARTESIAN_POINT('Origin',(5.8674,-3.74476680248583,3.74476680248583));
#17650=CARTESIAN_POINT('',(6.604,1.78435,-1.78435));
#17651=CARTESIAN_POINT('Origin',(54.0004,8.6995,0.));
#17652=CARTESIAN_POINT('Origin',(44.8564,8.6995,0.));
#17653=CARTESIAN_POINT('Origin',(38.1,6.06425,0.));
#17654=CARTESIAN_POINT('Origin',(3.048,5.55625,0.));
#17655=CARTESIAN_POINT('Origin',(2.6321124124205E-17,3.43630268540794E-34,
0.));
#17656=CARTESIAN_POINT('Origin',(6.604,3.5687,0.));
#17980=UNCERTAINTY_MEASURE_WITH_UNIT(LENGTH_MEASURE(0.01),#18007,
'DISTANCE_ACCURACY_VALUE',
'Maximum model space distance between geometric entities at asserted c
onnectivities');
#17986=UNCERTAINTY_MEASURE_WITH_UNIT(LENGTH_MEASURE(0.01),#18007,
'DISTANCE_ACCURACY_VALUE',
'Maximum model space distance between geometric entities at asserted c
onnectivities');
#18000=(
GEOMETRIC_REPRESENTATION_CONTEXT(3)
GLOBAL_UNCERTAINTY_ASSIGNED_CONTEXT((#17980))
GLOBAL_UNIT_ASSIGNED_CONTEXT((#18007,#18009,#18010))
REPRESENTATION_CONTEXT('','3D')
);
#18006=(
GEOMETRIC_REPRESENTATION_CONTEXT(3)
GLOBAL_UNCERTAINTY_ASSIGNED_CONTEXT((#17986))
GLOBAL_UNIT_ASSIGNED_CONTEXT((#18007,#18009,#18010))
REPRESENTATION_CONTEXT('','3D')
);
#18007=(
LENGTH_UNIT()
NAMED_UNIT(*)
SI_UNIT(.MILLI.,.METRE.)
);
#18009=(
NAMED_UNIT(*)
PLANE_ANGLE_UNIT()
SI_UNIT($,.RADIAN.)
);
#18010=(
NAMED_UNIT(*)
SI_UNIT($,.STERADIAN.)
SOLID_ANGLE_UNIT()
);
#18024=SHAPE_DEFINITION_REPRESENTATION(#18043,#18083);
#18043=PRODUCT_DEFINITION_SHAPE('',$,#18103);
#18083=SHAPE_REPRESENTATION('',(#10635),#18000);
#18089=PRODUCT_DEFINITION_CONTEXT('part definition',#18148,'design');
#18103=PRODUCT_DEFINITION('Swivel Stem','Swivel Stem',#18122,#18089);
#18122=PRODUCT_DEFINITION_FORMATION('',$,#18163);
#18148=APPLICATION_CONTEXT(
'Core Data for Automotive Mechanical Design Process');
#18149=PRODUCT_CONTEXT('part definition',#18148,'mechanical');
#18163=PRODUCT('Swivel Stem','Swivel Stem',$,(#18149));
#18170=PRESENTATION_STYLE_ASSIGNMENT((#18174));
#18174=SURFACE_STYLE_USAGE(.BOTH.,#18178);
#18178=SURFACE_SIDE_STYLE('',(#18182));
#18182=SURFACE_STYLE_FILL_AREA(#18186);
#18186=FILL_AREA_STYLE('Opaque(227,224,212)',(#18190));
#18190=FILL_AREA_STYLE_COLOUR('Opaque(227,224,212)',#18194);
#18194=COLOUR_RGB('Opaque(227,224,212)',0.890196078431372,0.87843137254902,
0.831372549019608);
ENDSEC;
END-ISO-10303-21;
